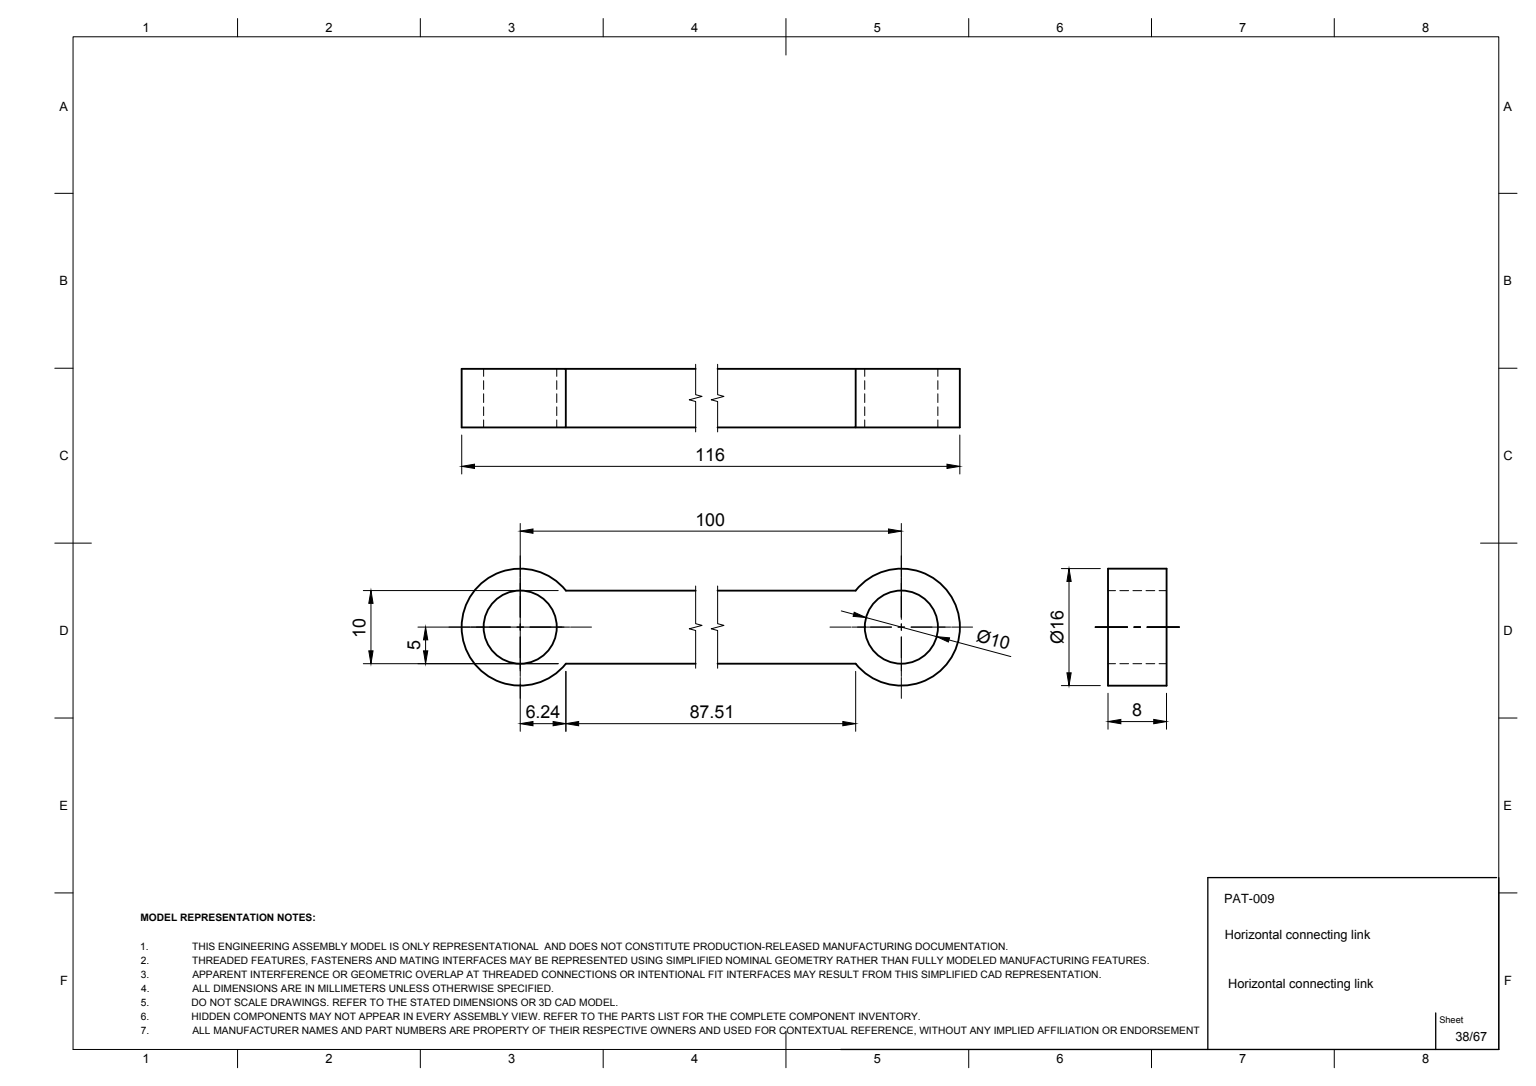
ISO-10303-21;
HEADER;
/* Generated by software containing ST-Developer
 * from STEP Tools, Inc. (www.steptools.com) 
 */

FILE_DESCRIPTION(
/* description */ ('Bell-crank linkage with push rods'),
/* implementation_level */ '2;1');

FILE_NAME(
/* name */ 'Horizontal connecting link.step',
/* time_stamp */ '2026-10-28T03:25:15-07:00',
/* author */ (''),
/* organization */ (''),
/* preprocessor_version */ 'ST-DEVELOPER v20.2',
/* originating_system */ 'Autodesk Translation Framework v15.17.0.0',
/* authorisation */ '');

FILE_SCHEMA (('AUTOMOTIVE_DESIGN { 1 0 10303 214 3 1 1 }'));
ENDSEC;

DATA;
#10=MECHANICAL_DESIGN_GEOMETRIC_PRESENTATION_REPRESENTATION('',(#643),#16678);
#527=SHAPE_REPRESENTATION_RELATIONSHIP('SRR','None',#16946,#581);
#581=ADVANCED_BREP_SHAPE_REPRESENTATION('',(#703),#16651);
#643=STYLED_ITEM('',(#17277),#703);
#703=MANIFOLD_SOLID_BREP('Body1',#8835);
#858=FACE_BOUND('',#2244,.T.);
#859=FACE_BOUND('',#2245,.T.);
#860=FACE_BOUND('',#2249,.T.);
#861=FACE_BOUND('',#2250,.T.);
#1143=PLANE('',#10167);
#1144=PLANE('',#10168);
#1145=PLANE('',#10170);
#1146=PLANE('',#10173);
#1584=FACE_OUTER_BOUND('',#2239,.T.);
#1585=FACE_OUTER_BOUND('',#2240,.T.);
#1586=FACE_OUTER_BOUND('',#2241,.T.);
#1587=FACE_OUTER_BOUND('',#2242,.T.);
#1588=FACE_OUTER_BOUND('',#2243,.T.);
#1589=FACE_OUTER_BOUND('',#2246,.T.);
#1590=FACE_OUTER_BOUND('',#2247,.T.);
#1591=FACE_OUTER_BOUND('',#2248,.T.);
#2239=EDGE_LOOP('',(#7335,#7336,#7337,#7338));
#2240=EDGE_LOOP('',(#7339,#7340,#7341,#7342));
#2241=EDGE_LOOP('',(#7343,#7344,#7345,#7346));
#2242=EDGE_LOOP('',(#7347,#7348,#7349,#7350));
#2243=EDGE_LOOP('',(#7351,#7352,#7353,#7354));
#2244=EDGE_LOOP('',(#7355));
#2245=EDGE_LOOP('',(#7356));
#2246=EDGE_LOOP('',(#7357,#7358,#7359,#7360));
#2247=EDGE_LOOP('',(#7361,#7362,#7363,#7364));
#2248=EDGE_LOOP('',(#7365,#7366,#7367,#7368));
#2249=EDGE_LOOP('',(#7369));
#2250=EDGE_LOOP('',(#7370));
#2880=LINE('',#15639,#3429);
#2881=LINE('',#15645,#3430);
#2882=LINE('',#15650,#3431);
#2883=LINE('',#15654,#3432);
#2884=LINE('',#15658,#3433);
#2885=LINE('',#15660,#3434);
#2886=LINE('',#15661,#3435);
#2887=LINE('',#15664,#3436);
#2888=LINE('',#15668,#3437);
#2889=LINE('',#15669,#3438);
#3429=VECTOR('',#12390,0.5);
#3430=VECTOR('',#12397,0.5);
#3431=VECTOR('',#12402,1.);
#3432=VECTOR('',#12405,1.);
#3433=VECTOR('',#12410,1.);
#3434=VECTOR('',#12411,1.);
#3435=VECTOR('',#12412,1.);
#3436=VECTOR('',#12415,1.);
#3437=VECTOR('',#12420,1.);
#3438=VECTOR('',#12421,1.);
#3955=CIRCLE('',#10159,0.5);
#3956=CIRCLE('',#10160,0.5);
#3957=CIRCLE('',#10162,0.5);
#3958=CIRCLE('',#10163,0.5);
#3959=CIRCLE('',#10165,0.800000000000001);
#3960=CIRCLE('',#10166,0.800000000000001);
#3961=CIRCLE('',#10169,0.8);
#3962=CIRCLE('',#10172,0.8);
#4590=VERTEX_POINT('',#15636);
#4591=VERTEX_POINT('',#15638);
#4592=VERTEX_POINT('',#15642);
#4593=VERTEX_POINT('',#15644);
#4594=VERTEX_POINT('',#15648);
#4595=VERTEX_POINT('',#15649);
#4596=VERTEX_POINT('',#15651);
#4597=VERTEX_POINT('',#15653);
#4598=VERTEX_POINT('',#15657);
#4599=VERTEX_POINT('',#15659);
#4600=VERTEX_POINT('',#15663);
#4601=VERTEX_POINT('',#15667);
#5545=EDGE_CURVE('',#4590,#4590,#3955,.T.);
#5546=EDGE_CURVE('',#4590,#4591,#2880,.T.);
#5547=EDGE_CURVE('',#4591,#4591,#3956,.T.);
#5548=EDGE_CURVE('',#4592,#4592,#3957,.T.);
#5549=EDGE_CURVE('',#4592,#4593,#2881,.T.);
#5550=EDGE_CURVE('',#4593,#4593,#3958,.T.);
#5551=EDGE_CURVE('',#4594,#4595,#2882,.T.);
#5552=EDGE_CURVE('',#4596,#4594,#3959,.T.);
#5553=EDGE_CURVE('',#4597,#4596,#2883,.T.);
#5554=EDGE_CURVE('',#4597,#4595,#3960,.T.);
#5555=EDGE_CURVE('',#4598,#4595,#2884,.T.);
#5556=EDGE_CURVE('',#4599,#4598,#2885,.T.);
#5557=EDGE_CURVE('',#4594,#4599,#2886,.T.);
#5558=EDGE_CURVE('',#4597,#4600,#2887,.T.);
#5559=EDGE_CURVE('',#4598,#4600,#3961,.T.);
#5560=EDGE_CURVE('',#4601,#4596,#2888,.T.);
#5561=EDGE_CURVE('',#4600,#4601,#2889,.T.);
#5562=EDGE_CURVE('',#4599,#4601,#3962,.T.);
#7335=ORIENTED_EDGE('',*,*,#5545,.F.);
#7336=ORIENTED_EDGE('',*,*,#5546,.T.);
#7337=ORIENTED_EDGE('',*,*,#5547,.F.);
#7338=ORIENTED_EDGE('',*,*,#5546,.F.);
#7339=ORIENTED_EDGE('',*,*,#5548,.F.);
#7340=ORIENTED_EDGE('',*,*,#5549,.T.);
#7341=ORIENTED_EDGE('',*,*,#5550,.F.);
#7342=ORIENTED_EDGE('',*,*,#5549,.F.);
#7343=ORIENTED_EDGE('',*,*,#5551,.F.);
#7344=ORIENTED_EDGE('',*,*,#5552,.F.);
#7345=ORIENTED_EDGE('',*,*,#5553,.F.);
#7346=ORIENTED_EDGE('',*,*,#5554,.T.);
#7347=ORIENTED_EDGE('',*,*,#5551,.T.);
#7348=ORIENTED_EDGE('',*,*,#5555,.F.);
#7349=ORIENTED_EDGE('',*,*,#5556,.F.);
#7350=ORIENTED_EDGE('',*,*,#5557,.F.);
#7351=ORIENTED_EDGE('',*,*,#5554,.F.);
#7352=ORIENTED_EDGE('',*,*,#5558,.T.);
#7353=ORIENTED_EDGE('',*,*,#5559,.F.);
#7354=ORIENTED_EDGE('',*,*,#5555,.T.);
#7355=ORIENTED_EDGE('',*,*,#5545,.T.);
#7356=ORIENTED_EDGE('',*,*,#5548,.T.);
#7357=ORIENTED_EDGE('',*,*,#5553,.T.);
#7358=ORIENTED_EDGE('',*,*,#5560,.F.);
#7359=ORIENTED_EDGE('',*,*,#5561,.F.);
#7360=ORIENTED_EDGE('',*,*,#5558,.F.);
#7361=ORIENTED_EDGE('',*,*,#5556,.T.);
#7362=ORIENTED_EDGE('',*,*,#5559,.T.);
#7363=ORIENTED_EDGE('',*,*,#5561,.T.);
#7364=ORIENTED_EDGE('',*,*,#5562,.F.);
#7365=ORIENTED_EDGE('',*,*,#5557,.T.);
#7366=ORIENTED_EDGE('',*,*,#5562,.T.);
#7367=ORIENTED_EDGE('',*,*,#5560,.T.);
#7368=ORIENTED_EDGE('',*,*,#5552,.T.);
#7369=ORIENTED_EDGE('',*,*,#5547,.T.);
#7370=ORIENTED_EDGE('',*,*,#5550,.T.);
#8194=CYLINDRICAL_SURFACE('',#10158,0.5);
#8195=CYLINDRICAL_SURFACE('',#10161,0.5);
#8196=CYLINDRICAL_SURFACE('',#10164,0.800000000000001);
#8197=CYLINDRICAL_SURFACE('',#10171,0.8);
#8609=ADVANCED_FACE('',(#1584),#8194,.F.);
#8610=ADVANCED_FACE('',(#1585),#8195,.F.);
#8611=ADVANCED_FACE('',(#1586),#8196,.T.);
#8612=ADVANCED_FACE('',(#1587),#1143,.T.);
#8613=ADVANCED_FACE('',(#1588,#858,#859),#1144,.F.);
#8614=ADVANCED_FACE('',(#1589),#1145,.T.);
#8615=ADVANCED_FACE('',(#1590),#8197,.T.);
#8616=ADVANCED_FACE('',(#1591,#860,#861),#1146,.T.);
#8835=CLOSED_SHELL('',(#8609,#8610,#8611,#8612,#8613,#8614,#8615,#8616));
#10157=AXIS2_PLACEMENT_3D('',#15634,#12384,#12385);
#10158=AXIS2_PLACEMENT_3D('',#15635,#12386,#12387);
#10159=AXIS2_PLACEMENT_3D('',#15637,#12388,#12389);
#10160=AXIS2_PLACEMENT_3D('',#15640,#12391,#12392);
#10161=AXIS2_PLACEMENT_3D('',#15641,#12393,#12394);
#10162=AXIS2_PLACEMENT_3D('',#15643,#12395,#12396);
#10163=AXIS2_PLACEMENT_3D('',#15646,#12398,#12399);
#10164=AXIS2_PLACEMENT_3D('',#15647,#12400,#12401);
#10165=AXIS2_PLACEMENT_3D('',#15652,#12403,#12404);
#10166=AXIS2_PLACEMENT_3D('',#15655,#12406,#12407);
#10167=AXIS2_PLACEMENT_3D('',#15656,#12408,#12409);
#10168=AXIS2_PLACEMENT_3D('',#15662,#12413,#12414);
#10169=AXIS2_PLACEMENT_3D('',#15665,#12416,#12417);
#10170=AXIS2_PLACEMENT_3D('',#15666,#12418,#12419);
#10171=AXIS2_PLACEMENT_3D('',#15670,#12422,#12423);
#10172=AXIS2_PLACEMENT_3D('',#15671,#12424,#12425);
#10173=AXIS2_PLACEMENT_3D('',#15672,#12426,#12427);
#12384=DIRECTION('axis',(0.,0.,1.));
#12385=DIRECTION('refdir',(1.,0.,0.));
#12386=DIRECTION('center_axis',(0.,0.,1.));
#12387=DIRECTION('ref_axis',(1.,0.,0.));
#12388=DIRECTION('center_axis',(0.,0.,1.));
#12389=DIRECTION('ref_axis',(1.,0.,0.));
#12390=DIRECTION('',(0.,0.,1.));
#12391=DIRECTION('center_axis',(0.,0.,-1.));
#12392=DIRECTION('ref_axis',(1.,0.,0.));
#12393=DIRECTION('center_axis',(0.,0.,1.));
#12394=DIRECTION('ref_axis',(1.,0.,0.));
#12395=DIRECTION('center_axis',(0.,0.,1.));
#12396=DIRECTION('ref_axis',(1.,0.,0.));
#12397=DIRECTION('',(0.,0.,1.));
#12398=DIRECTION('center_axis',(0.,0.,-1.));
#12399=DIRECTION('ref_axis',(1.,0.,0.));
#12400=DIRECTION('center_axis',(0.,0.,1.));
#12401=DIRECTION('ref_axis',(1.,0.,0.));
#12402=DIRECTION('',(0.,0.,-1.));
#12403=DIRECTION('center_axis',(0.,0.,1.));
#12404=DIRECTION('ref_axis',(1.,0.,0.));
#12405=DIRECTION('',(0.,0.,1.));
#12406=DIRECTION('center_axis',(0.,0.,1.));
#12407=DIRECTION('ref_axis',(1.,0.,0.));
#12408=DIRECTION('center_axis',(0.,1.,0.));
#12409=DIRECTION('ref_axis',(-1.,0.,0.));
#12410=DIRECTION('',(1.,0.,0.));
#12411=DIRECTION('',(0.,0.,-1.));
#12412=DIRECTION('',(-1.,0.,0.));
#12413=DIRECTION('center_axis',(0.,0.,1.));
#12414=DIRECTION('ref_axis',(1.,0.,0.));
#12415=DIRECTION('',(-1.,0.,0.));
#12416=DIRECTION('center_axis',(0.,0.,1.));
#12417=DIRECTION('ref_axis',(1.,0.,0.));
#12418=DIRECTION('center_axis',(0.,-1.,0.));
#12419=DIRECTION('ref_axis',(1.,0.,0.));
#12420=DIRECTION('',(1.,0.,0.));
#12421=DIRECTION('',(0.,0.,1.));
#12422=DIRECTION('center_axis',(0.,0.,1.));
#12423=DIRECTION('ref_axis',(-1.,1.22464679914735E-16,0.));
#12424=DIRECTION('center_axis',(0.,0.,1.));
#12425=DIRECTION('ref_axis',(1.,0.,0.));
#12426=DIRECTION('center_axis',(0.,0.,1.));
#12427=DIRECTION('ref_axis',(1.,0.,0.));
#15634=CARTESIAN_POINT('',(0.,0.,0.));
#15635=CARTESIAN_POINT('Origin',(0.,2.,8.7));
#15636=CARTESIAN_POINT('',(-0.5,2.,8.8));
#15637=CARTESIAN_POINT('Origin',(0.,2.,8.8));
#15638=CARTESIAN_POINT('',(-0.5,2.,9.6));
#15639=CARTESIAN_POINT('',(-0.5,2.,8.7));
#15640=CARTESIAN_POINT('Origin',(0.,2.,9.6));
#15641=CARTESIAN_POINT('Origin',(10.,2.,8.7));
#15642=CARTESIAN_POINT('',(9.5,2.,8.8));
#15643=CARTESIAN_POINT('Origin',(10.,2.,8.8));
#15644=CARTESIAN_POINT('',(9.5,2.,9.6));
#15645=CARTESIAN_POINT('',(9.5,2.,8.7));
#15646=CARTESIAN_POINT('Origin',(10.,2.,9.6));
#15647=CARTESIAN_POINT('Origin',(10.,2.,8.8));
#15648=CARTESIAN_POINT('',(9.37550020016016,2.5,9.6));
#15649=CARTESIAN_POINT('',(9.37550020016016,2.5,8.8));
#15650=CARTESIAN_POINT('',(9.37550020016016,2.5,8.8));
#15651=CARTESIAN_POINT('',(9.37550020016016,1.5,9.6));
#15652=CARTESIAN_POINT('Origin',(10.,2.,9.6));
#15653=CARTESIAN_POINT('',(9.37550020016016,1.5,8.8));
#15654=CARTESIAN_POINT('',(9.37550020016016,1.5,8.8));
#15655=CARTESIAN_POINT('Origin',(10.,2.,8.8));
#15656=CARTESIAN_POINT('Origin',(10.,2.5,8.8));
#15657=CARTESIAN_POINT('',(0.62449979983984,2.5,8.8));
#15658=CARTESIAN_POINT('',(0.,2.5,8.8));
#15659=CARTESIAN_POINT('',(0.62449979983984,2.5,9.6));
#15660=CARTESIAN_POINT('',(0.62449979983984,2.5,8.8));
#15661=CARTESIAN_POINT('',(0.,2.5,9.6));
#15662=CARTESIAN_POINT('Origin',(0.,2.,8.8));
#15663=CARTESIAN_POINT('',(0.62449979983984,1.5,8.8));
#15664=CARTESIAN_POINT('',(10.,1.5,8.8));
#15665=CARTESIAN_POINT('Origin',(0.,2.,8.8));
#15666=CARTESIAN_POINT('Origin',(0.,1.5,8.8));
#15667=CARTESIAN_POINT('',(0.62449979983984,1.5,9.6));
#15668=CARTESIAN_POINT('',(10.,1.5,9.6));
#15669=CARTESIAN_POINT('',(0.62449979983984,1.5,8.8));
#15670=CARTESIAN_POINT('Origin',(0.,2.,8.8));
#15671=CARTESIAN_POINT('Origin',(0.,2.,9.6));
#15672=CARTESIAN_POINT('Origin',(0.,2.,9.6));
#16587=UNCERTAINTY_MEASURE_WITH_UNIT(LENGTH_MEASURE(0.001),#16679,
'DISTANCE_ACCURACY_VALUE',
'Maximum model space distance between geometric entities at asserted c
onnectivities');
#16614=UNCERTAINTY_MEASURE_WITH_UNIT(LENGTH_MEASURE(0.001),#16679,
'DISTANCE_ACCURACY_VALUE',
'Maximum model space distance between geometric entities at asserted c
onnectivities');
#16651=(
GEOMETRIC_REPRESENTATION_CONTEXT(3)
GLOBAL_UNCERTAINTY_ASSIGNED_CONTEXT((#16587))
GLOBAL_UNIT_ASSIGNED_CONTEXT((#16679,#16681,#16682))
REPRESENTATION_CONTEXT('','3D')
);
#16678=(
GEOMETRIC_REPRESENTATION_CONTEXT(3)
GLOBAL_UNCERTAINTY_ASSIGNED_CONTEXT((#16614))
GLOBAL_UNIT_ASSIGNED_CONTEXT((#16679,#16681,#16682))
REPRESENTATION_CONTEXT('','3D')
);
#16679=(
LENGTH_UNIT()
NAMED_UNIT(*)
SI_UNIT(.CENTI.,.METRE.)
);
#16681=(
NAMED_UNIT(*)
PLANE_ANGLE_UNIT()
SI_UNIT($,.RADIAN.)
);
#16682=(
NAMED_UNIT(*)
SI_UNIT($,.STERADIAN.)
SOLID_ANGLE_UNIT()
);
#16719=SHAPE_DEFINITION_REPRESENTATION(#16787,#16946);
#16787=PRODUCT_DEFINITION_SHAPE('',$,#17010);
#16946=SHAPE_REPRESENTATION('',(#10157),#16651);
#16973=PRODUCT_DEFINITION_CONTEXT('part definition',#17164,'design');
#17010=PRODUCT_DEFINITION('Horizontal connecting link',
'Horizontal connecting link',#17073,#16973);
#17073=PRODUCT_DEFINITION_FORMATION('',$,#17202);
#17164=APPLICATION_CONTEXT(
'Core Data for Automotive Mechanical Design Process');
#17165=PRODUCT_CONTEXT('part definition',#17164,'mechanical');
#17202=PRODUCT('Horizontal connecting link',
'Horizontal connecting link','Horizontal connecting link',(#17165));
#17271=COLOUR_RGB('Light Blue',0.38,0.62,0.78);
#17272=FILL_AREA_STYLE_COLOUR('',#17271);
#17273=FILL_AREA_STYLE('',(#17272));
#17274=SURFACE_STYLE_FILL_AREA(#17273);
#17275=SURFACE_SIDE_STYLE('',(#17274));
#17276=SURFACE_STYLE_USAGE(.BOTH.,#17275);
#17277=PRESENTATION_STYLE_ASSIGNMENT((#17276));
ENDSEC;
END-ISO-10303-21;
